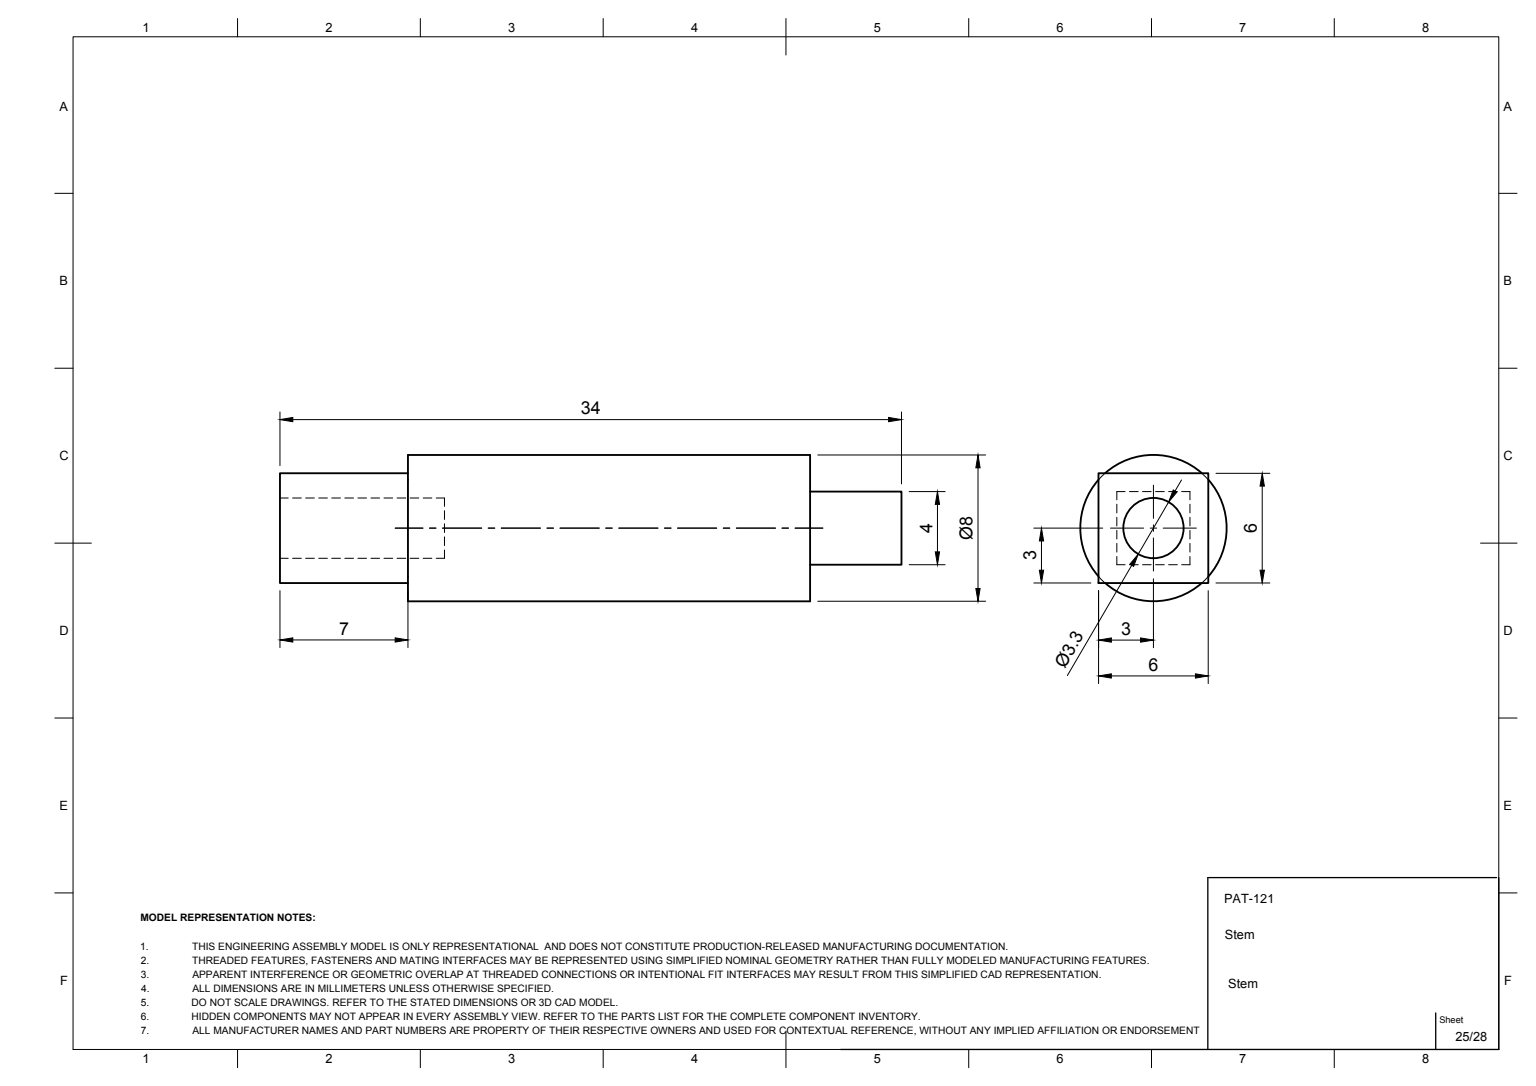
ISO-10303-21;
HEADER;
/* Generated by software containing ST-Developer
 * from STEP Tools, Inc. (www.steptools.com) 
 */

FILE_DESCRIPTION(
/* description */ ('Wall-mounted air drop station'),
/* implementation_level */ '2;1');

FILE_NAME(
/* name */ 'Stem.step',
/* time_stamp */ '2026-10-28T22:16:19-07:00',
/* author */ (''),
/* organization */ (''),
/* preprocessor_version */ 'ST-DEVELOPER v20.2',
/* originating_system */ 'Autodesk Translation Framework v15.17.0.0',
/* authorisation */ '');

FILE_SCHEMA (('AUTOMOTIVE_DESIGN { 1 0 10303 214 3 1 1 }'));
ENDSEC;

DATA;
#10=MECHANICAL_DESIGN_GEOMETRIC_PRESENTATION_REPRESENTATION('',(#368),#10517);
#310=SHAPE_REPRESENTATION_RELATIONSHIP('SRR','None',#10668,#339);
#339=ADVANCED_BREP_SHAPE_REPRESENTATION('',(#395),#10512);
#368=STYLED_ITEM('',(#10867),#395);
#395=MANIFOLD_SOLID_BREP('Body1',#5909);
#519=FACE_BOUND('',#1538,.T.);
#520=FACE_BOUND('',#1550,.T.);
#706=PLANE('',#6834);
#707=PLANE('',#6835);
#708=PLANE('',#6837);
#709=PLANE('',#6839);
#710=PLANE('',#6841);
#711=PLANE('',#6843);
#712=PLANE('',#6844);
#713=PLANE('',#6845);
#714=PLANE('',#6846);
#715=PLANE('',#6847);
#716=PLANE('',#6848);
#717=PLANE('',#6850);
#718=PLANE('',#6853);
#719=PLANE('',#6855);
#720=PLANE('',#6857);
#721=PLANE('',#6858);
#722=PLANE('',#6859);
#723=PLANE('',#6860);
#724=PLANE('',#6861);
#725=PLANE('',#6864);
#1052=FACE_OUTER_BOUND('',#1527,.T.);
#1053=FACE_OUTER_BOUND('',#1528,.T.);
#1054=FACE_OUTER_BOUND('',#1529,.T.);
#1055=FACE_OUTER_BOUND('',#1530,.T.);
#1056=FACE_OUTER_BOUND('',#1531,.T.);
#1057=FACE_OUTER_BOUND('',#1532,.T.);
#1058=FACE_OUTER_BOUND('',#1533,.T.);
#1059=FACE_OUTER_BOUND('',#1534,.T.);
#1060=FACE_OUTER_BOUND('',#1535,.T.);
#1061=FACE_OUTER_BOUND('',#1536,.T.);
#1062=FACE_OUTER_BOUND('',#1537,.T.);
#1063=FACE_OUTER_BOUND('',#1539,.T.);
#1064=FACE_OUTER_BOUND('',#1540,.T.);
#1065=FACE_OUTER_BOUND('',#1541,.T.);
#1066=FACE_OUTER_BOUND('',#1542,.T.);
#1067=FACE_OUTER_BOUND('',#1543,.T.);
#1068=FACE_OUTER_BOUND('',#1544,.T.);
#1069=FACE_OUTER_BOUND('',#1545,.T.);
#1070=FACE_OUTER_BOUND('',#1546,.T.);
#1071=FACE_OUTER_BOUND('',#1547,.T.);
#1072=FACE_OUTER_BOUND('',#1548,.T.);
#1073=FACE_OUTER_BOUND('',#1549,.T.);
#1527=EDGE_LOOP('',(#5195,#5196,#5197,#5198));
#1528=EDGE_LOOP('',(#5199));
#1529=EDGE_LOOP('',(#5200,#5201,#5202));
#1530=EDGE_LOOP('',(#5203,#5204,#5205));
#1531=EDGE_LOOP('',(#5206,#5207,#5208));
#1532=EDGE_LOOP('',(#5209,#5210,#5211));
#1533=EDGE_LOOP('',(#5212,#5213,#5214,#5215,#5216,#5217));
#1534=EDGE_LOOP('',(#5218,#5219,#5220,#5221,#5222,#5223));
#1535=EDGE_LOOP('',(#5224,#5225,#5226,#5227,#5228,#5229));
#1536=EDGE_LOOP('',(#5230,#5231,#5232,#5233,#5234,#5235));
#1537=EDGE_LOOP('',(#5236,#5237,#5238,#5239));
#1538=EDGE_LOOP('',(#5240));
#1539=EDGE_LOOP('',(#5241,#5242));
#1540=EDGE_LOOP('',(#5243,#5244,#5245));
#1541=EDGE_LOOP('',(#5246,#5247));
#1542=EDGE_LOOP('',(#5248,#5249));
#1543=EDGE_LOOP('',(#5250,#5251,#5252,#5253));
#1544=EDGE_LOOP('',(#5254,#5255,#5256,#5257));
#1545=EDGE_LOOP('',(#5258,#5259,#5260,#5261));
#1546=EDGE_LOOP('',(#5262,#5263,#5264,#5265));
#1547=EDGE_LOOP('',(#5266,#5267,#5268,#5269));
#1548=EDGE_LOOP('',(#5270,#5271,#5272,#5273,#5274,#5275,#5276,#5277,#5278,
#5279,#5280,#5281));
#1549=EDGE_LOOP('',(#5282));
#1550=EDGE_LOOP('',(#5283,#5284,#5285,#5286));
#1961=LINE('',#10193,#2425);
#1962=LINE('',#10201,#2426);
#1963=LINE('',#10202,#2427);
#1964=LINE('',#10208,#2428);
#1965=LINE('',#10209,#2429);
#1966=LINE('',#10215,#2430);
#1967=LINE('',#10216,#2431);
#1968=LINE('',#10222,#2432);
#1969=LINE('',#10223,#2433);
#1970=LINE('',#10225,#2434);
#1971=LINE('',#10227,#2435);
#1972=LINE('',#10229,#2436);
#1973=LINE('',#10230,#2437);
#1974=LINE('',#10232,#2438);
#1975=LINE('',#10234,#2439);
#1976=LINE('',#10235,#2440);
#1977=LINE('',#10237,#2441);
#1978=LINE('',#10239,#2442);
#1979=LINE('',#10240,#2443);
#1980=LINE('',#10242,#2444);
#1981=LINE('',#10243,#2445);
#1982=LINE('',#10258,#2446);
#1983=LINE('',#10260,#2447);
#1984=LINE('',#10262,#2448);
#1985=LINE('',#10263,#2449);
#1986=LINE('',#10266,#2450);
#1987=LINE('',#10268,#2451);
#1988=LINE('',#10269,#2452);
#1989=LINE('',#10272,#2453);
#1990=LINE('',#10274,#2454);
#1991=LINE('',#10275,#2455);
#1992=LINE('',#10277,#2456);
#1993=LINE('',#10278,#2457);
#1994=LINE('',#10282,#2458);
#2425=VECTOR('',#8489,0.165);
#2426=VECTOR('',#8498,1.);
#2427=VECTOR('',#8499,1.);
#2428=VECTOR('',#8504,1.);
#2429=VECTOR('',#8505,1.);
#2430=VECTOR('',#8510,1.);
#2431=VECTOR('',#8511,1.);
#2432=VECTOR('',#8516,1.);
#2433=VECTOR('',#8517,1.);
#2434=VECTOR('',#8520,1.);
#2435=VECTOR('',#8521,1.);
#2436=VECTOR('',#8522,1.);
#2437=VECTOR('',#8523,1.);
#2438=VECTOR('',#8526,1.);
#2439=VECTOR('',#8527,1.);
#2440=VECTOR('',#8528,1.);
#2441=VECTOR('',#8531,1.);
#2442=VECTOR('',#8532,1.);
#2443=VECTOR('',#8533,1.);
#2444=VECTOR('',#8536,1.);
#2445=VECTOR('',#8537,1.);
#2446=VECTOR('',#8560,1.);
#2447=VECTOR('',#8561,1.);
#2448=VECTOR('',#8562,1.);
#2449=VECTOR('',#8563,1.);
#2450=VECTOR('',#8566,1.);
#2451=VECTOR('',#8567,1.);
#2452=VECTOR('',#8568,1.);
#2453=VECTOR('',#8571,1.);
#2454=VECTOR('',#8572,1.);
#2455=VECTOR('',#8573,1.);
#2456=VECTOR('',#8576,1.);
#2457=VECTOR('',#8577,1.);
#2458=VECTOR('',#8582,0.4);
#2742=CIRCLE('',#6832,0.165);
#2743=CIRCLE('',#6833,0.165);
#2744=CIRCLE('',#6836,0.4);
#2745=CIRCLE('',#6838,0.4);
#2746=CIRCLE('',#6840,0.4);
#2747=CIRCLE('',#6842,0.4);
#2748=CIRCLE('',#6849,0.4);
#2749=CIRCLE('',#6851,0.4);
#2750=CIRCLE('',#6852,0.4);
#2751=CIRCLE('',#6854,0.4);
#2752=CIRCLE('',#6856,0.4);
#2753=CIRCLE('',#6863,0.4);
#3169=VERTEX_POINT('',#10190);
#3170=VERTEX_POINT('',#10192);
#3171=VERTEX_POINT('',#10197);
#3172=VERTEX_POINT('',#10198);
#3173=VERTEX_POINT('',#10200);
#3174=VERTEX_POINT('',#10204);
#3175=VERTEX_POINT('',#10205);
#3176=VERTEX_POINT('',#10207);
#3177=VERTEX_POINT('',#10211);
#3178=VERTEX_POINT('',#10212);
#3179=VERTEX_POINT('',#10214);
#3180=VERTEX_POINT('',#10218);
#3181=VERTEX_POINT('',#10219);
#3182=VERTEX_POINT('',#10221);
#3183=VERTEX_POINT('',#10226);
#3184=VERTEX_POINT('',#10228);
#3185=VERTEX_POINT('',#10233);
#3186=VERTEX_POINT('',#10238);
#3187=VERTEX_POINT('',#10248);
#3188=VERTEX_POINT('',#10256);
#3189=VERTEX_POINT('',#10257);
#3190=VERTEX_POINT('',#10259);
#3191=VERTEX_POINT('',#10261);
#3192=VERTEX_POINT('',#10265);
#3193=VERTEX_POINT('',#10267);
#3194=VERTEX_POINT('',#10271);
#3195=VERTEX_POINT('',#10273);
#3196=VERTEX_POINT('',#10281);
#3855=EDGE_CURVE('',#3169,#3169,#2742,.T.);
#3856=EDGE_CURVE('',#3169,#3170,#1961,.T.);
#3857=EDGE_CURVE('',#3170,#3170,#2743,.T.);
#3858=EDGE_CURVE('',#3171,#3172,#2744,.T.);
#3859=EDGE_CURVE('',#3173,#3172,#1962,.T.);
#3860=EDGE_CURVE('',#3171,#3173,#1963,.T.);
#3861=EDGE_CURVE('',#3174,#3175,#2745,.T.);
#3862=EDGE_CURVE('',#3176,#3175,#1964,.T.);
#3863=EDGE_CURVE('',#3174,#3176,#1965,.T.);
#3864=EDGE_CURVE('',#3177,#3178,#2746,.T.);
#3865=EDGE_CURVE('',#3179,#3178,#1966,.T.);
#3866=EDGE_CURVE('',#3177,#3179,#1967,.T.);
#3867=EDGE_CURVE('',#3180,#3181,#2747,.T.);
#3868=EDGE_CURVE('',#3182,#3181,#1968,.T.);
#3869=EDGE_CURVE('',#3180,#3182,#1969,.T.);
#3870=EDGE_CURVE('',#3171,#3181,#1970,.T.);
#3871=EDGE_CURVE('',#3173,#3183,#1971,.T.);
#3872=EDGE_CURVE('',#3184,#3183,#1972,.T.);
#3873=EDGE_CURVE('',#3182,#3184,#1973,.T.);
#3874=EDGE_CURVE('',#3180,#3178,#1974,.T.);
#3875=EDGE_CURVE('',#3185,#3184,#1975,.T.);
#3876=EDGE_CURVE('',#3179,#3185,#1976,.T.);
#3877=EDGE_CURVE('',#3177,#3175,#1977,.T.);
#3878=EDGE_CURVE('',#3186,#3185,#1978,.T.);
#3879=EDGE_CURVE('',#3176,#3186,#1979,.T.);
#3880=EDGE_CURVE('',#3174,#3172,#1980,.T.);
#3881=EDGE_CURVE('',#3183,#3186,#1981,.T.);
#3882=EDGE_CURVE('',#3175,#3177,#2748,.T.);
#3883=EDGE_CURVE('',#3172,#3187,#2749,.T.);
#3884=EDGE_CURVE('',#3187,#3174,#2750,.T.);
#3885=EDGE_CURVE('',#3181,#3171,#2751,.T.);
#3886=EDGE_CURVE('',#3178,#3180,#2752,.T.);
#3887=EDGE_CURVE('',#3188,#3189,#1982,.T.);
#3888=EDGE_CURVE('',#3189,#3190,#1983,.T.);
#3889=EDGE_CURVE('',#3191,#3190,#1984,.T.);
#3890=EDGE_CURVE('',#3188,#3191,#1985,.T.);
#3891=EDGE_CURVE('',#3192,#3188,#1986,.T.);
#3892=EDGE_CURVE('',#3193,#3191,#1987,.T.);
#3893=EDGE_CURVE('',#3192,#3193,#1988,.T.);
#3894=EDGE_CURVE('',#3194,#3192,#1989,.T.);
#3895=EDGE_CURVE('',#3195,#3193,#1990,.T.);
#3896=EDGE_CURVE('',#3194,#3195,#1991,.T.);
#3897=EDGE_CURVE('',#3189,#3194,#1992,.T.);
#3898=EDGE_CURVE('',#3190,#3195,#1993,.T.);
#3899=EDGE_CURVE('',#3187,#3196,#1994,.T.);
#3900=EDGE_CURVE('',#3196,#3196,#2753,.T.);
#5195=ORIENTED_EDGE('',*,*,#3855,.F.);
#5196=ORIENTED_EDGE('',*,*,#3856,.T.);
#5197=ORIENTED_EDGE('',*,*,#3857,.F.);
#5198=ORIENTED_EDGE('',*,*,#3856,.F.);
#5199=ORIENTED_EDGE('',*,*,#3855,.T.);
#5200=ORIENTED_EDGE('',*,*,#3858,.T.);
#5201=ORIENTED_EDGE('',*,*,#3859,.F.);
#5202=ORIENTED_EDGE('',*,*,#3860,.F.);
#5203=ORIENTED_EDGE('',*,*,#3861,.T.);
#5204=ORIENTED_EDGE('',*,*,#3862,.F.);
#5205=ORIENTED_EDGE('',*,*,#3863,.F.);
#5206=ORIENTED_EDGE('',*,*,#3864,.T.);
#5207=ORIENTED_EDGE('',*,*,#3865,.F.);
#5208=ORIENTED_EDGE('',*,*,#3866,.F.);
#5209=ORIENTED_EDGE('',*,*,#3867,.T.);
#5210=ORIENTED_EDGE('',*,*,#3868,.F.);
#5211=ORIENTED_EDGE('',*,*,#3869,.F.);
#5212=ORIENTED_EDGE('',*,*,#3868,.T.);
#5213=ORIENTED_EDGE('',*,*,#3870,.F.);
#5214=ORIENTED_EDGE('',*,*,#3860,.T.);
#5215=ORIENTED_EDGE('',*,*,#3871,.T.);
#5216=ORIENTED_EDGE('',*,*,#3872,.F.);
#5217=ORIENTED_EDGE('',*,*,#3873,.F.);
#5218=ORIENTED_EDGE('',*,*,#3865,.T.);
#5219=ORIENTED_EDGE('',*,*,#3874,.F.);
#5220=ORIENTED_EDGE('',*,*,#3869,.T.);
#5221=ORIENTED_EDGE('',*,*,#3873,.T.);
#5222=ORIENTED_EDGE('',*,*,#3875,.F.);
#5223=ORIENTED_EDGE('',*,*,#3876,.F.);
#5224=ORIENTED_EDGE('',*,*,#3862,.T.);
#5225=ORIENTED_EDGE('',*,*,#3877,.F.);
#5226=ORIENTED_EDGE('',*,*,#3866,.T.);
#5227=ORIENTED_EDGE('',*,*,#3876,.T.);
#5228=ORIENTED_EDGE('',*,*,#3878,.F.);
#5229=ORIENTED_EDGE('',*,*,#3879,.F.);
#5230=ORIENTED_EDGE('',*,*,#3859,.T.);
#5231=ORIENTED_EDGE('',*,*,#3880,.F.);
#5232=ORIENTED_EDGE('',*,*,#3863,.T.);
#5233=ORIENTED_EDGE('',*,*,#3879,.T.);
#5234=ORIENTED_EDGE('',*,*,#3881,.F.);
#5235=ORIENTED_EDGE('',*,*,#3871,.F.);
#5236=ORIENTED_EDGE('',*,*,#3881,.T.);
#5237=ORIENTED_EDGE('',*,*,#3878,.T.);
#5238=ORIENTED_EDGE('',*,*,#3875,.T.);
#5239=ORIENTED_EDGE('',*,*,#3872,.T.);
#5240=ORIENTED_EDGE('',*,*,#3857,.T.);
#5241=ORIENTED_EDGE('',*,*,#3877,.T.);
#5242=ORIENTED_EDGE('',*,*,#3882,.T.);
#5243=ORIENTED_EDGE('',*,*,#3880,.T.);
#5244=ORIENTED_EDGE('',*,*,#3883,.T.);
#5245=ORIENTED_EDGE('',*,*,#3884,.T.);
#5246=ORIENTED_EDGE('',*,*,#3870,.T.);
#5247=ORIENTED_EDGE('',*,*,#3885,.T.);
#5248=ORIENTED_EDGE('',*,*,#3874,.T.);
#5249=ORIENTED_EDGE('',*,*,#3886,.T.);
#5250=ORIENTED_EDGE('',*,*,#3887,.T.);
#5251=ORIENTED_EDGE('',*,*,#3888,.T.);
#5252=ORIENTED_EDGE('',*,*,#3889,.F.);
#5253=ORIENTED_EDGE('',*,*,#3890,.F.);
#5254=ORIENTED_EDGE('',*,*,#3891,.T.);
#5255=ORIENTED_EDGE('',*,*,#3890,.T.);
#5256=ORIENTED_EDGE('',*,*,#3892,.F.);
#5257=ORIENTED_EDGE('',*,*,#3893,.F.);
#5258=ORIENTED_EDGE('',*,*,#3894,.T.);
#5259=ORIENTED_EDGE('',*,*,#3893,.T.);
#5260=ORIENTED_EDGE('',*,*,#3895,.F.);
#5261=ORIENTED_EDGE('',*,*,#3896,.F.);
#5262=ORIENTED_EDGE('',*,*,#3897,.T.);
#5263=ORIENTED_EDGE('',*,*,#3896,.T.);
#5264=ORIENTED_EDGE('',*,*,#3898,.F.);
#5265=ORIENTED_EDGE('',*,*,#3888,.F.);
#5266=ORIENTED_EDGE('',*,*,#3897,.F.);
#5267=ORIENTED_EDGE('',*,*,#3887,.F.);
#5268=ORIENTED_EDGE('',*,*,#3891,.F.);
#5269=ORIENTED_EDGE('',*,*,#3894,.F.);
#5270=ORIENTED_EDGE('',*,*,#3883,.F.);
#5271=ORIENTED_EDGE('',*,*,#3858,.F.);
#5272=ORIENTED_EDGE('',*,*,#3885,.F.);
#5273=ORIENTED_EDGE('',*,*,#3867,.F.);
#5274=ORIENTED_EDGE('',*,*,#3886,.F.);
#5275=ORIENTED_EDGE('',*,*,#3864,.F.);
#5276=ORIENTED_EDGE('',*,*,#3882,.F.);
#5277=ORIENTED_EDGE('',*,*,#3861,.F.);
#5278=ORIENTED_EDGE('',*,*,#3884,.F.);
#5279=ORIENTED_EDGE('',*,*,#3899,.T.);
#5280=ORIENTED_EDGE('',*,*,#3900,.T.);
#5281=ORIENTED_EDGE('',*,*,#3899,.F.);
#5282=ORIENTED_EDGE('',*,*,#3900,.F.);
#5283=ORIENTED_EDGE('',*,*,#3889,.T.);
#5284=ORIENTED_EDGE('',*,*,#3898,.T.);
#5285=ORIENTED_EDGE('',*,*,#3895,.T.);
#5286=ORIENTED_EDGE('',*,*,#3892,.T.);
#5522=CYLINDRICAL_SURFACE('',#6831,0.165);
#5523=CYLINDRICAL_SURFACE('',#6862,0.4);
#5825=ADVANCED_FACE('',(#1052),#5522,.F.);
#5826=ADVANCED_FACE('',(#1053),#706,.T.);
#5827=ADVANCED_FACE('',(#1054),#707,.F.);
#5828=ADVANCED_FACE('',(#1055),#708,.F.);
#5829=ADVANCED_FACE('',(#1056),#709,.F.);
#5830=ADVANCED_FACE('',(#1057),#710,.F.);
#5831=ADVANCED_FACE('',(#1058),#711,.T.);
#5832=ADVANCED_FACE('',(#1059),#712,.T.);
#5833=ADVANCED_FACE('',(#1060),#713,.T.);
#5834=ADVANCED_FACE('',(#1061),#714,.T.);
#5835=ADVANCED_FACE('',(#1062,#519),#715,.T.);
#5836=ADVANCED_FACE('',(#1063),#716,.T.);
#5837=ADVANCED_FACE('',(#1064),#717,.T.);
#5838=ADVANCED_FACE('',(#1065),#718,.T.);
#5839=ADVANCED_FACE('',(#1066),#719,.T.);
#5840=ADVANCED_FACE('',(#1067),#720,.T.);
#5841=ADVANCED_FACE('',(#1068),#721,.T.);
#5842=ADVANCED_FACE('',(#1069),#722,.T.);
#5843=ADVANCED_FACE('',(#1070),#723,.T.);
#5844=ADVANCED_FACE('',(#1071),#724,.F.);
#5845=ADVANCED_FACE('',(#1072),#5523,.T.);
#5846=ADVANCED_FACE('',(#1073,#520),#725,.F.);
#5909=CLOSED_SHELL('',(#5825,#5826,#5827,#5828,#5829,#5830,#5831,#5832,
#5833,#5834,#5835,#5836,#5837,#5838,#5839,#5840,#5841,#5842,#5843,#5844,
#5845,#5846));
#6830=AXIS2_PLACEMENT_3D('',#10188,#8483,#8484);
#6831=AXIS2_PLACEMENT_3D('',#10189,#8485,#8486);
#6832=AXIS2_PLACEMENT_3D('',#10191,#8487,#8488);
#6833=AXIS2_PLACEMENT_3D('',#10194,#8490,#8491);
#6834=AXIS2_PLACEMENT_3D('',#10195,#8492,#8493);
#6835=AXIS2_PLACEMENT_3D('',#10196,#8494,#8495);
#6836=AXIS2_PLACEMENT_3D('',#10199,#8496,#8497);
#6837=AXIS2_PLACEMENT_3D('',#10203,#8500,#8501);
#6838=AXIS2_PLACEMENT_3D('',#10206,#8502,#8503);
#6839=AXIS2_PLACEMENT_3D('',#10210,#8506,#8507);
#6840=AXIS2_PLACEMENT_3D('',#10213,#8508,#8509);
#6841=AXIS2_PLACEMENT_3D('',#10217,#8512,#8513);
#6842=AXIS2_PLACEMENT_3D('',#10220,#8514,#8515);
#6843=AXIS2_PLACEMENT_3D('',#10224,#8518,#8519);
#6844=AXIS2_PLACEMENT_3D('',#10231,#8524,#8525);
#6845=AXIS2_PLACEMENT_3D('',#10236,#8529,#8530);
#6846=AXIS2_PLACEMENT_3D('',#10241,#8534,#8535);
#6847=AXIS2_PLACEMENT_3D('',#10244,#8538,#8539);
#6848=AXIS2_PLACEMENT_3D('',#10245,#8540,#8541);
#6849=AXIS2_PLACEMENT_3D('',#10246,#8542,#8543);
#6850=AXIS2_PLACEMENT_3D('',#10247,#8544,#8545);
#6851=AXIS2_PLACEMENT_3D('',#10249,#8546,#8547);
#6852=AXIS2_PLACEMENT_3D('',#10250,#8548,#8549);
#6853=AXIS2_PLACEMENT_3D('',#10251,#8550,#8551);
#6854=AXIS2_PLACEMENT_3D('',#10252,#8552,#8553);
#6855=AXIS2_PLACEMENT_3D('',#10253,#8554,#8555);
#6856=AXIS2_PLACEMENT_3D('',#10254,#8556,#8557);
#6857=AXIS2_PLACEMENT_3D('',#10255,#8558,#8559);
#6858=AXIS2_PLACEMENT_3D('',#10264,#8564,#8565);
#6859=AXIS2_PLACEMENT_3D('',#10270,#8569,#8570);
#6860=AXIS2_PLACEMENT_3D('',#10276,#8574,#8575);
#6861=AXIS2_PLACEMENT_3D('',#10279,#8578,#8579);
#6862=AXIS2_PLACEMENT_3D('',#10280,#8580,#8581);
#6863=AXIS2_PLACEMENT_3D('',#10283,#8583,#8584);
#6864=AXIS2_PLACEMENT_3D('',#10284,#8585,#8586);
#8483=DIRECTION('axis',(0.,0.,1.));
#8484=DIRECTION('refdir',(1.,0.,0.));
#8485=DIRECTION('center_axis',(0.,0.,1.));
#8486=DIRECTION('ref_axis',(1.,0.,0.));
#8487=DIRECTION('center_axis',(0.,0.,1.));
#8488=DIRECTION('ref_axis',(1.,0.,0.));
#8489=DIRECTION('',(0.,0.,1.));
#8490=DIRECTION('center_axis',(0.,0.,-1.));
#8491=DIRECTION('ref_axis',(1.,0.,0.));
#8492=DIRECTION('center_axis',(0.,0.,1.));
#8493=DIRECTION('ref_axis',(1.,0.,0.));
#8494=DIRECTION('center_axis',(0.,0.,1.));
#8495=DIRECTION('ref_axis',(1.,0.,0.));
#8496=DIRECTION('center_axis',(0.,0.,1.));
#8497=DIRECTION('ref_axis',(1.,0.,0.));
#8498=DIRECTION('',(0.,-1.,0.));
#8499=DIRECTION('',(-1.,0.,0.));
#8500=DIRECTION('center_axis',(0.,0.,1.));
#8501=DIRECTION('ref_axis',(1.,0.,0.));
#8502=DIRECTION('center_axis',(0.,0.,1.));
#8503=DIRECTION('ref_axis',(1.,0.,0.));
#8504=DIRECTION('',(1.,0.,0.));
#8505=DIRECTION('',(0.,-1.,0.));
#8506=DIRECTION('center_axis',(0.,0.,1.));
#8507=DIRECTION('ref_axis',(1.,0.,0.));
#8508=DIRECTION('center_axis',(0.,0.,1.));
#8509=DIRECTION('ref_axis',(1.,0.,0.));
#8510=DIRECTION('',(0.,1.,0.));
#8511=DIRECTION('',(1.,0.,0.));
#8512=DIRECTION('center_axis',(0.,0.,1.));
#8513=DIRECTION('ref_axis',(1.,0.,0.));
#8514=DIRECTION('center_axis',(0.,0.,1.));
#8515=DIRECTION('ref_axis',(1.,0.,0.));
#8516=DIRECTION('',(-1.,0.,0.));
#8517=DIRECTION('',(0.,1.,0.));
#8518=DIRECTION('center_axis',(0.,1.,0.));
#8519=DIRECTION('ref_axis',(-1.,0.,0.));
#8520=DIRECTION('',(1.,0.,0.));
#8521=DIRECTION('',(0.,0.,1.));
#8522=DIRECTION('',(-1.,0.,0.));
#8523=DIRECTION('',(0.,0.,1.));
#8524=DIRECTION('center_axis',(1.,0.,0.));
#8525=DIRECTION('ref_axis',(0.,1.,0.));
#8526=DIRECTION('',(0.,-1.,0.));
#8527=DIRECTION('',(0.,1.,0.));
#8528=DIRECTION('',(0.,0.,1.));
#8529=DIRECTION('center_axis',(0.,-1.,0.));
#8530=DIRECTION('ref_axis',(1.,0.,0.));
#8531=DIRECTION('',(-1.,0.,0.));
#8532=DIRECTION('',(1.,0.,0.));
#8533=DIRECTION('',(0.,0.,1.));
#8534=DIRECTION('center_axis',(-1.,0.,0.));
#8535=DIRECTION('ref_axis',(0.,-1.,0.));
#8536=DIRECTION('',(0.,1.,0.));
#8537=DIRECTION('',(0.,-1.,0.));
#8538=DIRECTION('center_axis',(0.,0.,1.));
#8539=DIRECTION('ref_axis',(1.,0.,0.));
#8540=DIRECTION('center_axis',(0.,0.,1.));
#8541=DIRECTION('ref_axis',(1.,0.,0.));
#8542=DIRECTION('center_axis',(0.,0.,1.));
#8543=DIRECTION('ref_axis',(1.,0.,0.));
#8544=DIRECTION('center_axis',(0.,0.,1.));
#8545=DIRECTION('ref_axis',(1.,0.,0.));
#8546=DIRECTION('center_axis',(0.,0.,1.));
#8547=DIRECTION('ref_axis',(1.,0.,0.));
#8548=DIRECTION('center_axis',(0.,0.,1.));
#8549=DIRECTION('ref_axis',(1.,0.,0.));
#8550=DIRECTION('center_axis',(0.,0.,1.));
#8551=DIRECTION('ref_axis',(1.,0.,0.));
#8552=DIRECTION('center_axis',(0.,0.,1.));
#8553=DIRECTION('ref_axis',(1.,0.,0.));
#8554=DIRECTION('center_axis',(0.,0.,1.));
#8555=DIRECTION('ref_axis',(1.,0.,0.));
#8556=DIRECTION('center_axis',(0.,0.,1.));
#8557=DIRECTION('ref_axis',(1.,0.,0.));
#8558=DIRECTION('center_axis',(0.,1.,0.));
#8559=DIRECTION('ref_axis',(-1.,0.,0.));
#8560=DIRECTION('',(-1.,0.,0.));
#8561=DIRECTION('',(0.,0.,1.));
#8562=DIRECTION('',(-1.,0.,0.));
#8563=DIRECTION('',(0.,0.,1.));
#8564=DIRECTION('center_axis',(1.,0.,0.));
#8565=DIRECTION('ref_axis',(0.,1.,0.));
#8566=DIRECTION('',(0.,1.,0.));
#8567=DIRECTION('',(0.,1.,0.));
#8568=DIRECTION('',(0.,0.,1.));
#8569=DIRECTION('center_axis',(0.,-1.,0.));
#8570=DIRECTION('ref_axis',(1.,0.,0.));
#8571=DIRECTION('',(1.,0.,0.));
#8572=DIRECTION('',(1.,0.,0.));
#8573=DIRECTION('',(0.,0.,1.));
#8574=DIRECTION('center_axis',(-1.,0.,0.));
#8575=DIRECTION('ref_axis',(0.,-1.,0.));
#8576=DIRECTION('',(0.,-1.,0.));
#8577=DIRECTION('',(0.,-1.,0.));
#8578=DIRECTION('center_axis',(0.,0.,1.));
#8579=DIRECTION('ref_axis',(1.,0.,0.));
#8580=DIRECTION('center_axis',(0.,0.,1.));
#8581=DIRECTION('ref_axis',(1.,0.,0.));
#8582=DIRECTION('',(0.,0.,-1.));
#8583=DIRECTION('center_axis',(0.,0.,1.));
#8584=DIRECTION('ref_axis',(1.,0.,0.));
#8585=DIRECTION('center_axis',(0.,0.,1.));
#8586=DIRECTION('ref_axis',(1.,0.,0.));
#10188=CARTESIAN_POINT('',(0.,0.,0.));
#10189=CARTESIAN_POINT('Origin',(0.,0.,8.5));
#10190=CARTESIAN_POINT('',(-0.165,-2.02066721859313E-17,8.5));
#10191=CARTESIAN_POINT('Origin',(0.,0.,8.5));
#10192=CARTESIAN_POINT('',(-0.165,2.02066721859313E-17,9.4));
#10193=CARTESIAN_POINT('',(-0.165,-2.02066721859313E-17,8.5));
#10194=CARTESIAN_POINT('Origin',(0.,0.,9.4));
#10195=CARTESIAN_POINT('Origin',(0.,0.,8.5));
#10196=CARTESIAN_POINT('Origin',(0.,0.,8.7));
#10197=CARTESIAN_POINT('',(-0.264575131106459,0.3,8.7));
#10198=CARTESIAN_POINT('',(-0.3,0.264575131106459,8.7));
#10199=CARTESIAN_POINT('Origin',(0.,0.,8.7));
#10200=CARTESIAN_POINT('',(-0.3,0.3,8.7));
#10201=CARTESIAN_POINT('',(-0.3,0.3,8.7));
#10202=CARTESIAN_POINT('',(0.3,0.3,8.7));
#10203=CARTESIAN_POINT('Origin',(0.,0.,8.7));
#10204=CARTESIAN_POINT('',(-0.3,-0.264575131106459,8.7));
#10205=CARTESIAN_POINT('',(-0.264575131106459,-0.3,8.7));
#10206=CARTESIAN_POINT('Origin',(0.,0.,8.7));
#10207=CARTESIAN_POINT('',(-0.3,-0.3,8.7));
#10208=CARTESIAN_POINT('',(-0.3,-0.3,8.7));
#10209=CARTESIAN_POINT('',(-0.3,0.3,8.7));
#10210=CARTESIAN_POINT('Origin',(0.,0.,8.7));
#10211=CARTESIAN_POINT('',(0.264575131106459,-0.3,8.7));
#10212=CARTESIAN_POINT('',(0.3,-0.264575131106459,8.7));
#10213=CARTESIAN_POINT('Origin',(0.,0.,8.7));
#10214=CARTESIAN_POINT('',(0.3,-0.3,8.7));
#10215=CARTESIAN_POINT('',(0.3,-0.3,8.7));
#10216=CARTESIAN_POINT('',(-0.3,-0.3,8.7));
#10217=CARTESIAN_POINT('Origin',(0.,0.,8.7));
#10218=CARTESIAN_POINT('',(0.3,0.264575131106459,8.7));
#10219=CARTESIAN_POINT('',(0.264575131106459,0.3,8.7));
#10220=CARTESIAN_POINT('Origin',(0.,0.,8.7));
#10221=CARTESIAN_POINT('',(0.3,0.3,8.7));
#10222=CARTESIAN_POINT('',(0.3,0.3,8.7));
#10223=CARTESIAN_POINT('',(0.3,-0.3,8.7));
#10224=CARTESIAN_POINT('Origin',(0.3,0.3,8.7));
#10225=CARTESIAN_POINT('',(0.15,0.3,8.7));
#10226=CARTESIAN_POINT('',(-0.3,0.3,9.4));
#10227=CARTESIAN_POINT('',(-0.3,0.3,8.7));
#10228=CARTESIAN_POINT('',(0.3,0.3,9.4));
#10229=CARTESIAN_POINT('',(0.3,0.3,9.4));
#10230=CARTESIAN_POINT('',(0.3,0.3,8.7));
#10231=CARTESIAN_POINT('Origin',(0.3,-0.3,8.7));
#10232=CARTESIAN_POINT('',(0.3,-0.15,8.7));
#10233=CARTESIAN_POINT('',(0.3,-0.3,9.4));
#10234=CARTESIAN_POINT('',(0.3,-0.3,9.4));
#10235=CARTESIAN_POINT('',(0.3,-0.3,8.7));
#10236=CARTESIAN_POINT('Origin',(-0.3,-0.3,8.7));
#10237=CARTESIAN_POINT('',(-0.15,-0.3,8.7));
#10238=CARTESIAN_POINT('',(-0.3,-0.3,9.4));
#10239=CARTESIAN_POINT('',(-0.3,-0.3,9.4));
#10240=CARTESIAN_POINT('',(-0.3,-0.3,8.7));
#10241=CARTESIAN_POINT('Origin',(-0.3,0.3,8.7));
#10242=CARTESIAN_POINT('',(-0.3,0.15,8.7));
#10243=CARTESIAN_POINT('',(-0.3,0.3,9.4));
#10244=CARTESIAN_POINT('Origin',(0.,0.,9.4));
#10245=CARTESIAN_POINT('Origin',(0.,0.,8.7));
#10246=CARTESIAN_POINT('Origin',(0.,0.,8.7));
#10247=CARTESIAN_POINT('Origin',(0.,0.,8.7));
#10248=CARTESIAN_POINT('',(-0.4,-4.89858719658941E-17,8.7));
#10249=CARTESIAN_POINT('Origin',(0.,0.,8.7));
#10250=CARTESIAN_POINT('Origin',(0.,0.,8.7));
#10251=CARTESIAN_POINT('Origin',(0.,0.,8.7));
#10252=CARTESIAN_POINT('Origin',(0.,0.,8.7));
#10253=CARTESIAN_POINT('Origin',(0.,0.,8.7));
#10254=CARTESIAN_POINT('Origin',(0.,0.,8.7));
#10255=CARTESIAN_POINT('Origin',(0.2,0.2,6.));
#10256=CARTESIAN_POINT('',(0.2,0.2,6.));
#10257=CARTESIAN_POINT('',(-0.2,0.2,6.));
#10258=CARTESIAN_POINT('',(0.2,0.2,6.));
#10259=CARTESIAN_POINT('',(-0.2,0.2,6.5));
#10260=CARTESIAN_POINT('',(-0.2,0.2,6.));
#10261=CARTESIAN_POINT('',(0.2,0.2,6.5));
#10262=CARTESIAN_POINT('',(0.1,0.2,6.5));
#10263=CARTESIAN_POINT('',(0.2,0.2,6.));
#10264=CARTESIAN_POINT('Origin',(0.2,-0.2,6.));
#10265=CARTESIAN_POINT('',(0.2,-0.2,6.));
#10266=CARTESIAN_POINT('',(0.2,-0.2,6.));
#10267=CARTESIAN_POINT('',(0.2,-0.2,6.5));
#10268=CARTESIAN_POINT('',(0.2,-0.1,6.5));
#10269=CARTESIAN_POINT('',(0.2,-0.2,6.));
#10270=CARTESIAN_POINT('Origin',(-0.2,-0.2,6.));
#10271=CARTESIAN_POINT('',(-0.2,-0.2,6.));
#10272=CARTESIAN_POINT('',(-0.2,-0.2,6.));
#10273=CARTESIAN_POINT('',(-0.2,-0.2,6.5));
#10274=CARTESIAN_POINT('',(-0.1,-0.2,6.5));
#10275=CARTESIAN_POINT('',(-0.2,-0.2,6.));
#10276=CARTESIAN_POINT('Origin',(-0.2,0.2,6.));
#10277=CARTESIAN_POINT('',(-0.2,0.2,6.));
#10278=CARTESIAN_POINT('',(-0.2,0.1,6.5));
#10279=CARTESIAN_POINT('Origin',(0.,0.,6.));
#10280=CARTESIAN_POINT('Origin',(0.,0.,6.5));
#10281=CARTESIAN_POINT('',(-0.4,-4.89858719658941E-17,6.5));
#10282=CARTESIAN_POINT('',(-0.4,-4.89858719658941E-17,6.5));
#10283=CARTESIAN_POINT('Origin',(0.,0.,6.5));
#10284=CARTESIAN_POINT('Origin',(0.,0.,6.5));
#10479=UNCERTAINTY_MEASURE_WITH_UNIT(LENGTH_MEASURE(0.001),#10518,
'DISTANCE_ACCURACY_VALUE',
'Maximum model space distance between geometric entities at asserted c
onnectivities');
#10484=UNCERTAINTY_MEASURE_WITH_UNIT(LENGTH_MEASURE(0.001),#10518,
'DISTANCE_ACCURACY_VALUE',
'Maximum model space distance between geometric entities at asserted c
onnectivities');
#10512=(
GEOMETRIC_REPRESENTATION_CONTEXT(3)
GLOBAL_UNCERTAINTY_ASSIGNED_CONTEXT((#10479))
GLOBAL_UNIT_ASSIGNED_CONTEXT((#10518,#10520,#10521))
REPRESENTATION_CONTEXT('','3D')
);
#10517=(
GEOMETRIC_REPRESENTATION_CONTEXT(3)
GLOBAL_UNCERTAINTY_ASSIGNED_CONTEXT((#10484))
GLOBAL_UNIT_ASSIGNED_CONTEXT((#10518,#10520,#10521))
REPRESENTATION_CONTEXT('','3D')
);
#10518=(
LENGTH_UNIT()
NAMED_UNIT(*)
SI_UNIT(.CENTI.,.METRE.)
);
#10520=(
NAMED_UNIT(*)
PLANE_ANGLE_UNIT()
SI_UNIT($,.RADIAN.)
);
#10521=(
NAMED_UNIT(*)
SI_UNIT($,.STERADIAN.)
SOLID_ANGLE_UNIT()
);
#10549=SHAPE_DEFINITION_REPRESENTATION(#10628,#10668);
#10628=PRODUCT_DEFINITION_SHAPE('',$,#10701);
#10668=SHAPE_REPRESENTATION('',(#6830),#10512);
#10673=PRODUCT_DEFINITION_CONTEXT('part definition',#10771,'design');
#10701=PRODUCT_DEFINITION('Stem','Stem',#10733,#10673);
#10733=PRODUCT_DEFINITION_FORMATION('',$,#10800);
#10771=APPLICATION_CONTEXT(
'Core Data for Automotive Mechanical Design Process');
#10772=PRODUCT_CONTEXT('part definition',#10771,'mechanical');
#10800=PRODUCT('Stem','Stem','Stem',(#10772));
#10861=COLOUR_RGB('Sky Blue',0.24,0.69,0.87);
#10862=FILL_AREA_STYLE_COLOUR('',#10861);
#10863=FILL_AREA_STYLE('',(#10862));
#10864=SURFACE_STYLE_FILL_AREA(#10863);
#10865=SURFACE_SIDE_STYLE('',(#10864));
#10866=SURFACE_STYLE_USAGE(.BOTH.,#10865);
#10867=PRESENTATION_STYLE_ASSIGNMENT((#10866));
ENDSEC;
END-ISO-10303-21;
